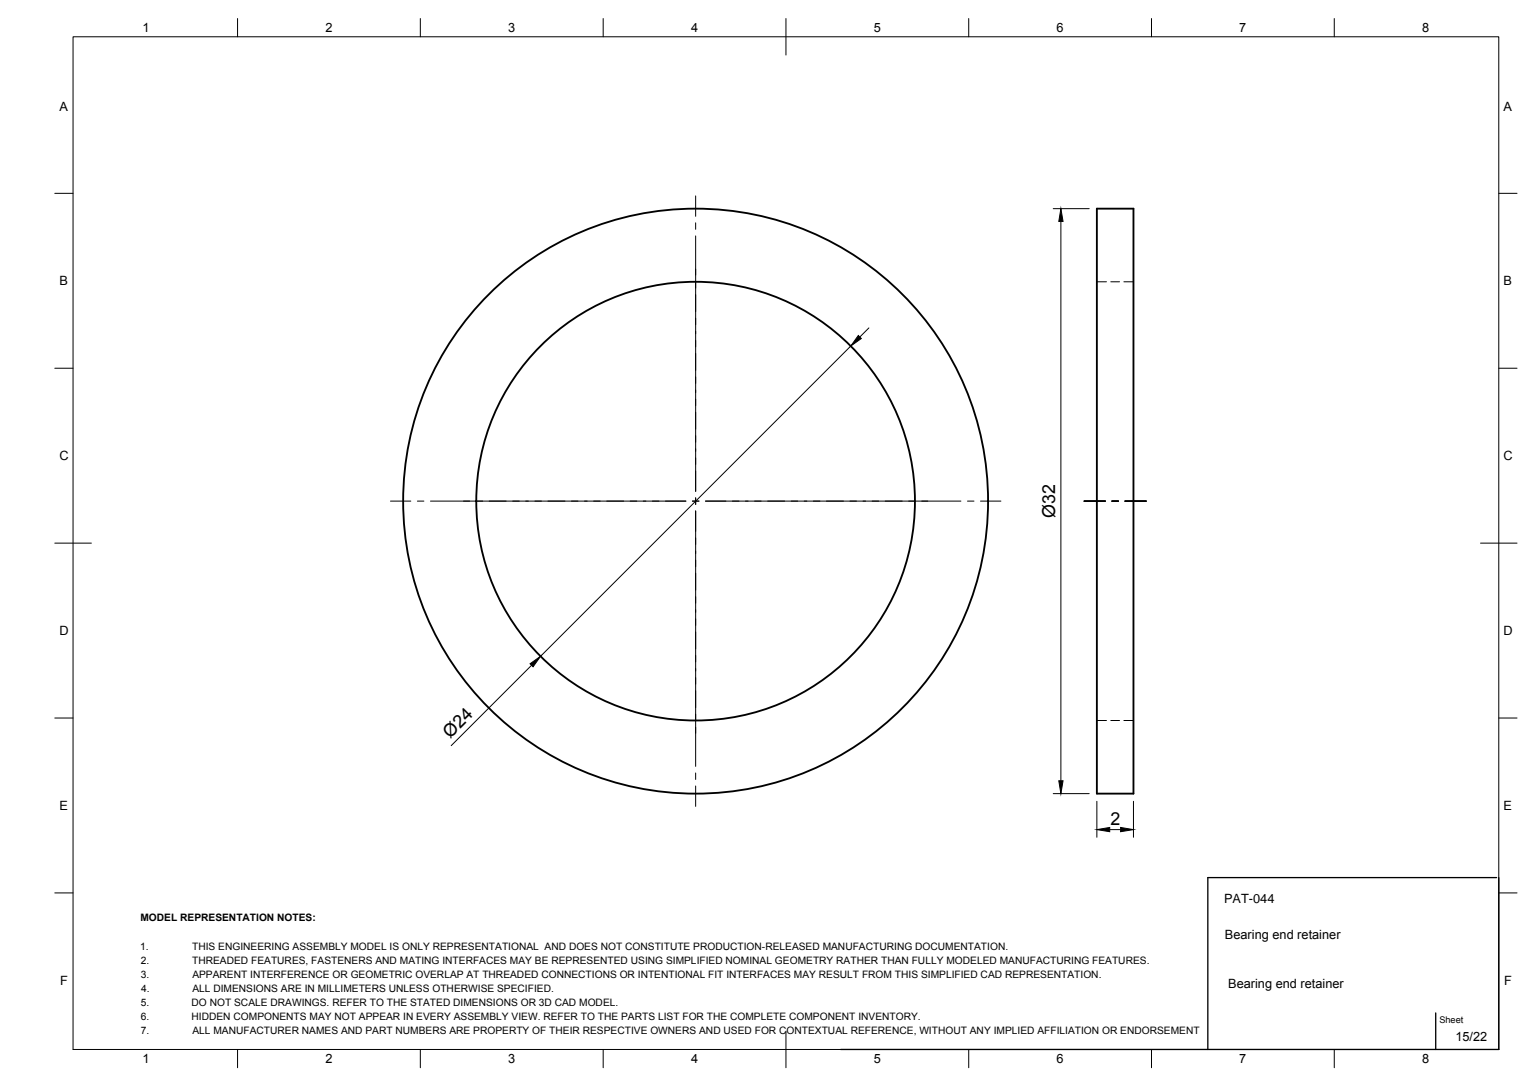
ISO-10303-21;
HEADER;
/* Generated by software containing ST-Developer
 * from STEP Tools, Inc. (www.steptools.com) 
 */

FILE_DESCRIPTION(
/* description */ ('Four-wheel beam trolley'),
/* implementation_level */ '2;1');

FILE_NAME(
/* name */ 'Bearing end retainer.step',
/* time_stamp */ '2026-10-29T16:22:06-07:00',
/* author */ (''),
/* organization */ (''),
/* preprocessor_version */ 'ST-DEVELOPER v20.2',
/* originating_system */ 'Autodesk Translation Framework v15.17.0.0',
/* authorisation */ '');

FILE_SCHEMA (('AUTOMOTIVE_DESIGN { 1 0 10303 214 3 1 1 }'));
ENDSEC;

DATA;
#10=MECHANICAL_DESIGN_GEOMETRIC_PRESENTATION_REPRESENTATION('',(#301),#4777);
#260=SHAPE_REPRESENTATION_RELATIONSHIP('SRR','None',#4891,#277);
#277=ADVANCED_BREP_SHAPE_REPRESENTATION('',(#323),#4776);
#301=STYLED_ITEM('',(#5056),#323);
#323=MANIFOLD_SOLID_BREP('Body1',#2390);
#363=FACE_BOUND('',#774,.T.);
#364=FACE_BOUND('',#776,.T.);
#440=PLANE('',#2920);
#441=PLANE('',#2921);
#585=FACE_OUTER_BOUND('',#771,.T.);
#586=FACE_OUTER_BOUND('',#772,.T.);
#587=FACE_OUTER_BOUND('',#773,.T.);
#588=FACE_OUTER_BOUND('',#775,.T.);
#771=EDGE_LOOP('',(#2163,#2164,#2165,#2166));
#772=EDGE_LOOP('',(#2167,#2168,#2169,#2170));
#773=EDGE_LOOP('',(#2171));
#774=EDGE_LOOP('',(#2172));
#775=EDGE_LOOP('',(#2173));
#776=EDGE_LOOP('',(#2174));
#898=LINE('',#4714,#1021);
#899=LINE('',#4720,#1022);
#1021=VECTOR('',#3727,1.2);
#1022=VECTOR('',#3734,1.6);
#1157=CIRCLE('',#2915,1.2);
#1158=CIRCLE('',#2916,1.2);
#1159=CIRCLE('',#2918,1.6);
#1160=CIRCLE('',#2919,1.6);
#1346=VERTEX_POINT('',#4711);
#1347=VERTEX_POINT('',#4713);
#1348=VERTEX_POINT('',#4717);
#1349=VERTEX_POINT('',#4719);
#1619=EDGE_CURVE('',#1346,#1346,#1157,.T.);
#1620=EDGE_CURVE('',#1346,#1347,#898,.T.);
#1621=EDGE_CURVE('',#1347,#1347,#1158,.T.);
#1622=EDGE_CURVE('',#1348,#1348,#1159,.T.);
#1623=EDGE_CURVE('',#1348,#1349,#899,.T.);
#1624=EDGE_CURVE('',#1349,#1349,#1160,.T.);
#2163=ORIENTED_EDGE('',*,*,#1619,.F.);
#2164=ORIENTED_EDGE('',*,*,#1620,.T.);
#2165=ORIENTED_EDGE('',*,*,#1621,.T.);
#2166=ORIENTED_EDGE('',*,*,#1620,.F.);
#2167=ORIENTED_EDGE('',*,*,#1622,.F.);
#2168=ORIENTED_EDGE('',*,*,#1623,.T.);
#2169=ORIENTED_EDGE('',*,*,#1624,.T.);
#2170=ORIENTED_EDGE('',*,*,#1623,.F.);
#2171=ORIENTED_EDGE('',*,*,#1622,.T.);
#2172=ORIENTED_EDGE('',*,*,#1619,.T.);
#2173=ORIENTED_EDGE('',*,*,#1624,.F.);
#2174=ORIENTED_EDGE('',*,*,#1621,.F.);
#2216=CYLINDRICAL_SURFACE('',#2914,1.2);
#2217=CYLINDRICAL_SURFACE('',#2917,1.6);
#2361=ADVANCED_FACE('',(#585),#2216,.F.);
#2362=ADVANCED_FACE('',(#586),#2217,.T.);
#2363=ADVANCED_FACE('',(#587,#363),#440,.T.);
#2364=ADVANCED_FACE('',(#588,#364),#441,.F.);
#2390=CLOSED_SHELL('',(#2361,#2362,#2363,#2364));
#2913=AXIS2_PLACEMENT_3D('',#4709,#3721,#3722);
#2914=AXIS2_PLACEMENT_3D('',#4710,#3723,#3724);
#2915=AXIS2_PLACEMENT_3D('',#4712,#3725,#3726);
#2916=AXIS2_PLACEMENT_3D('',#4715,#3728,#3729);
#2917=AXIS2_PLACEMENT_3D('',#4716,#3730,#3731);
#2918=AXIS2_PLACEMENT_3D('',#4718,#3732,#3733);
#2919=AXIS2_PLACEMENT_3D('',#4721,#3735,#3736);
#2920=AXIS2_PLACEMENT_3D('',#4722,#3737,#3738);
#2921=AXIS2_PLACEMENT_3D('',#4723,#3739,#3740);
#3721=DIRECTION('axis',(0.,0.,1.));
#3722=DIRECTION('refdir',(1.,0.,0.));
#3723=DIRECTION('center_axis',(0.,1.,0.));
#3724=DIRECTION('ref_axis',(1.,0.,0.));
#3725=DIRECTION('center_axis',(0.,-1.,0.));
#3726=DIRECTION('ref_axis',(1.,0.,0.));
#3727=DIRECTION('',(0.,-1.,0.));
#3728=DIRECTION('center_axis',(0.,-1.,0.));
#3729=DIRECTION('ref_axis',(1.,0.,0.));
#3730=DIRECTION('center_axis',(0.,1.,0.));
#3731=DIRECTION('ref_axis',(1.,0.,0.));
#3732=DIRECTION('center_axis',(0.,1.,0.));
#3733=DIRECTION('ref_axis',(1.,0.,0.));
#3734=DIRECTION('',(0.,-1.,0.));
#3735=DIRECTION('center_axis',(0.,1.,0.));
#3736=DIRECTION('ref_axis',(1.,0.,0.));
#3737=DIRECTION('center_axis',(0.,1.,0.));
#3738=DIRECTION('ref_axis',(1.,0.,0.));
#3739=DIRECTION('center_axis',(0.,1.,0.));
#3740=DIRECTION('ref_axis',(1.,0.,0.));
#4709=CARTESIAN_POINT('',(0.,0.,0.));
#4710=CARTESIAN_POINT('Origin',(0.,1.1,3.5));
#4711=CARTESIAN_POINT('',(-1.2,1.3,3.5));
#4712=CARTESIAN_POINT('Origin',(0.,1.3,3.5));
#4713=CARTESIAN_POINT('',(-1.2,1.1,3.5));
#4714=CARTESIAN_POINT('',(-1.2,1.1,3.5));
#4715=CARTESIAN_POINT('Origin',(0.,1.1,3.5));
#4716=CARTESIAN_POINT('Origin',(0.,1.1,3.5));
#4717=CARTESIAN_POINT('',(-1.6,1.3,3.5));
#4718=CARTESIAN_POINT('Origin',(0.,1.3,3.5));
#4719=CARTESIAN_POINT('',(-1.6,1.1,3.5));
#4720=CARTESIAN_POINT('',(-1.6,1.1,3.5));
#4721=CARTESIAN_POINT('Origin',(0.,1.1,3.5));
#4722=CARTESIAN_POINT('Origin',(0.,1.3,3.5));
#4723=CARTESIAN_POINT('Origin',(0.,1.1,3.5));
#4754=UNCERTAINTY_MEASURE_WITH_UNIT(LENGTH_MEASURE(0.001),#4778,
'DISTANCE_ACCURACY_VALUE',
'Maximum model space distance between geometric entities at asserted c
onnectivities');
#4755=UNCERTAINTY_MEASURE_WITH_UNIT(LENGTH_MEASURE(0.001),#4778,
'DISTANCE_ACCURACY_VALUE',
'Maximum model space distance between geometric entities at asserted c
onnectivities');
#4776=(
GEOMETRIC_REPRESENTATION_CONTEXT(3)
GLOBAL_UNCERTAINTY_ASSIGNED_CONTEXT((#4754))
GLOBAL_UNIT_ASSIGNED_CONTEXT((#4778,#4780,#4781))
REPRESENTATION_CONTEXT('','3D')
);
#4777=(
GEOMETRIC_REPRESENTATION_CONTEXT(3)
GLOBAL_UNCERTAINTY_ASSIGNED_CONTEXT((#4755))
GLOBAL_UNIT_ASSIGNED_CONTEXT((#4778,#4780,#4781))
REPRESENTATION_CONTEXT('','3D')
);
#4778=(
LENGTH_UNIT()
NAMED_UNIT(*)
SI_UNIT(.CENTI.,.METRE.)
);
#4780=(
NAMED_UNIT(*)
PLANE_ANGLE_UNIT()
SI_UNIT($,.RADIAN.)
);
#4781=(
NAMED_UNIT(*)
SI_UNIT($,.STERADIAN.)
SOLID_ANGLE_UNIT()
);
#4802=SHAPE_DEFINITION_REPRESENTATION(#4860,#4891);
#4860=PRODUCT_DEFINITION_SHAPE('',$,#4913);
#4891=SHAPE_REPRESENTATION('',(#2913),#4776);
#4892=PRODUCT_DEFINITION_CONTEXT('part definition',#4957,'design');
#4913=PRODUCT_DEFINITION('Bearing end retainer','Bearing end retainer',
#4934,#4892);
#4934=PRODUCT_DEFINITION_FORMATION('',$,#4979);
#4957=APPLICATION_CONTEXT(
'Core Data for Automotive Mechanical Design Process');
#4958=PRODUCT_CONTEXT('part definition',#4957,'mechanical');
#4979=PRODUCT('Bearing end retainer','Bearing end retainer',
'Bearing end retainer',(#4958));
#5050=COLOUR_RGB('Grey',0.48,0.52,0.57);
#5051=FILL_AREA_STYLE_COLOUR('',#5050);
#5052=FILL_AREA_STYLE('',(#5051));
#5053=SURFACE_STYLE_FILL_AREA(#5052);
#5054=SURFACE_SIDE_STYLE('',(#5053));
#5055=SURFACE_STYLE_USAGE(.BOTH.,#5054);
#5056=PRESENTATION_STYLE_ASSIGNMENT((#5055));
ENDSEC;
END-ISO-10303-21;
